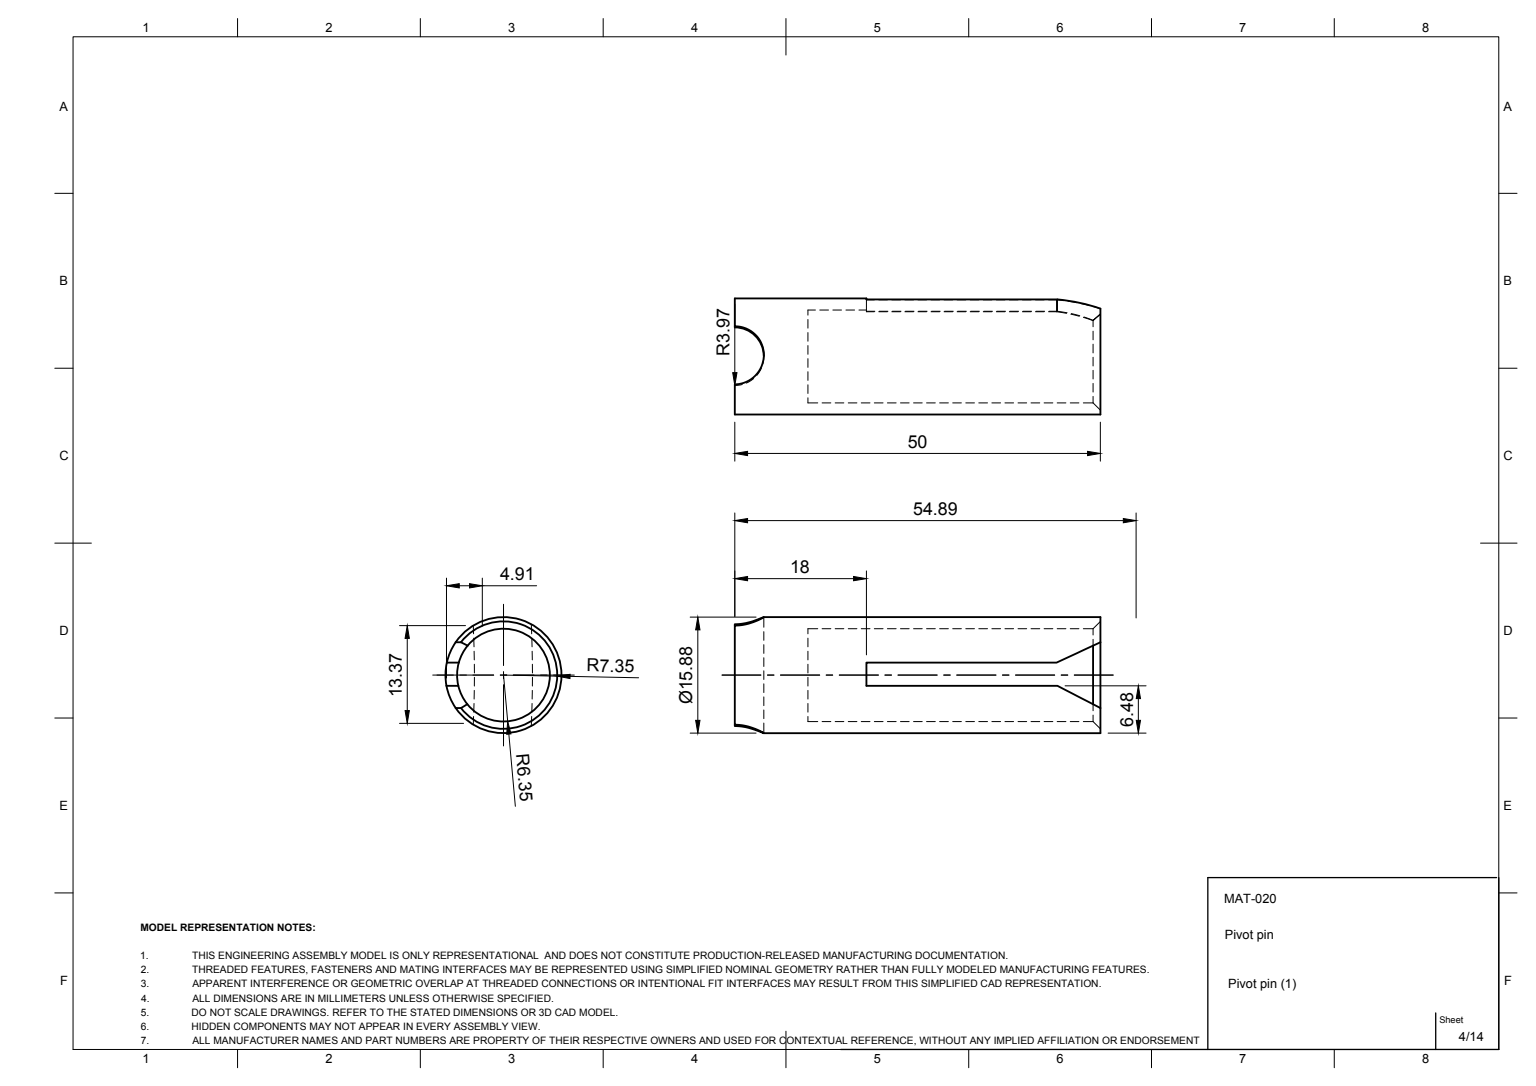
ISO-10303-21;
HEADER;
/* Generated by software containing ST-Developer
 * from STEP Tools, Inc. (www.steptools.com) 
 */

FILE_DESCRIPTION(
/* description */ ('STEP AP214'),
/* implementation_level */ '2;1');

FILE_NAME(
/* name */ 'Pivot Pin.step',
/* time_stamp */ '2026-11-14T06:20:50-08:00',
/* author */ (''),
/* organization */ (''),
/* preprocessor_version */ 'ST-DEVELOPER v20.2',
/* originating_system */ 'Autodesk Translation Framework v15.17.0.0',
/* authorisation */ '');

FILE_SCHEMA (('AUTOMOTIVE_DESIGN { 1 0 10303 214 3 1 1 }'));
ENDSEC;

DATA;
#10=MECHANICAL_DESIGN_GEOMETRIC_PRESENTATION_REPRESENTATION('',(#967),#20658);
#115=CONICAL_SURFACE('',#4073,6.35000000000001,0.785398163397456);
#148=ELLIPSE('',#4079,13.8289418104825,6.34999999998296);
#149=ELLIPSE('',#4080,15.0727020037017,6.35000000001005);
#150=ELLIPSE('',#4086,17.286177263089,7.93749999997138);
#151=ELLIPSE('',#4088,18.840877504683,7.93750000004892);
#292=(
BOUNDED_CURVE()
B_SPLINE_CURVE(2,(#20498,#20499,#20500),.UNSPECIFIED.,.F.,.F.)
B_SPLINE_CURVE_WITH_KNOTS((3,3),(0.0183343553427957,0.042559607390491),
 .UNSPECIFIED.)
CURVE()
GEOMETRIC_REPRESENTATION_ITEM()
RATIONAL_B_SPLINE_CURVE((1.12800823010849,1.2118132350172,1.29359962909812))
REPRESENTATION_ITEM('')
);
#293=(
BOUNDED_CURVE()
B_SPLINE_CURVE(2,(#20503,#20504,#20505),.UNSPECIFIED.,.F.,.F.)
B_SPLINE_CURVE_WITH_KNOTS((3,3),(-0.061743756665462,-0.0265578055647394),
 .UNSPECIFIED.)
CURVE()
GEOMETRIC_REPRESENTATION_ITEM()
RATIONAL_B_SPLINE_CURVE((1.28203378876711,1.20432016972132,1.12358878740287))
REPRESENTATION_ITEM('')
);
#391=B_SPLINE_CURVE_WITH_KNOTS('',3,(#20526,#20527,#20528,#20529,#20530,
#20531,#20532,#20533,#20534,#20535,#20536,#20537,#20538,#20539,#20540,#20541,
#20542,#20543,#20544,#20545,#20546,#20547),.UNSPECIFIED.,.F.,.F.,(4,2,2,
2,2,2,2,2,2,2,4),(1.27322512801248,1.33474273520392,1.47506259652504,1.63354487754016,
1.7891729428134,1.93308978701607,2.07370553081328,2.22765816465705,2.39186406247873,
2.46887047840366,2.54509076244393),.UNSPECIFIED.);
#392=B_SPLINE_CURVE_WITH_KNOTS('',3,(#20567,#20568,#20569,#20570,#20571,
#20572,#20573,#20574,#20575,#20576,#20577,#20578,#20579,#20580,#20581,#20582,
#20583,#20584,#20585,#20586),.UNSPECIFIED.,.F.,.F.,(4,2,2,2,2,2,2,2,2,4),
(0.,0.133781719517655,0.281821942641468,0.447759981880601,0.597114390464313,
0.737248938214622,0.881128826876862,1.04037144466368,1.19403526065854,1.27322512801215),
 .UNSPECIFIED.);
#439=PLANE('',#4091);
#440=PLANE('',#4093);
#441=PLANE('',#4095);
#442=PLANE('',#4096);
#443=PLANE('',#4097);
#444=PLANE('',#4098);
#445=PLANE('',#4099);
#446=PLANE('',#4100);
#447=PLANE('',#4102);
#629=LINE('',#20510,#822);
#630=LINE('',#20514,#823);
#631=LINE('',#20519,#824);
#632=LINE('',#20551,#825);
#633=LINE('',#20557,#826);
#634=LINE('',#20561,#827);
#635=LINE('',#20592,#828);
#636=LINE('',#20593,#829);
#637=LINE('',#20595,#830);
#638=LINE('',#20596,#831);
#639=LINE('',#20598,#832);
#640=LINE('',#20600,#833);
#822=VECTOR('',#4874,6.35000000000001);
#823=VECTOR('',#4877,1000.);
#824=VECTOR('',#4882,1000.);
#825=VECTOR('',#4891,7.93750000000001);
#826=VECTOR('',#4896,1000.);
#827=VECTOR('',#4899,1000.);
#828=VECTOR('',#4916,1000.);
#829=VECTOR('',#4917,1000.);
#830=VECTOR('',#4920,1000.);
#831=VECTOR('',#4921,1000.);
#832=VECTOR('',#4924,1000.);
#833=VECTOR('',#4927,1000.);
#930=CYLINDRICAL_SURFACE('',#4076,6.35000000000001);
#931=CYLINDRICAL_SURFACE('',#4082,7.93750000000001);
#943=SHAPE_REPRESENTATION_RELATIONSHIP('SRR','None',#20727,#955);
#955=ADVANCED_BREP_SHAPE_REPRESENTATION('',(#979),#20657);
#967=STYLED_ITEM('',(#20786),#979);
#979=MANIFOLD_SOLID_BREP('Body1',#3662);
#1176=FACE_OUTER_BOUND('',#1408,.T.);
#1177=FACE_OUTER_BOUND('',#1409,.T.);
#1178=FACE_OUTER_BOUND('',#1410,.T.);
#1179=FACE_OUTER_BOUND('',#1411,.T.);
#1180=FACE_OUTER_BOUND('',#1412,.T.);
#1181=FACE_OUTER_BOUND('',#1413,.T.);
#1182=FACE_OUTER_BOUND('',#1414,.T.);
#1183=FACE_OUTER_BOUND('',#1415,.T.);
#1184=FACE_OUTER_BOUND('',#1416,.T.);
#1185=FACE_OUTER_BOUND('',#1417,.T.);
#1186=FACE_OUTER_BOUND('',#1418,.T.);
#1187=FACE_OUTER_BOUND('',#1419,.T.);
#1188=FACE_OUTER_BOUND('',#1420,.T.);
#1408=EDGE_LOOP('',(#3374,#3375,#3376,#3377));
#1409=EDGE_LOOP('',(#3378,#3379,#3380,#3381,#3382,#3383,#3384,#3385,#3386,
#3387));
#1410=EDGE_LOOP('',(#3388,#3389,#3390,#3391,#3392,#3393,#3394,#3395,#3396,
#3397,#3398,#3399,#3400,#3401));
#1411=EDGE_LOOP('',(#3402,#3403,#3404));
#1412=EDGE_LOOP('',(#3405,#3406));
#1413=EDGE_LOOP('',(#3407,#3408,#3409,#3410,#3411));
#1414=EDGE_LOOP('',(#3412,#3413,#3414,#3415));
#1415=EDGE_LOOP('',(#3416,#3417,#3418,#3419,#3420));
#1416=EDGE_LOOP('',(#3421,#3422,#3423,#3424));
#1417=EDGE_LOOP('',(#3425,#3426,#3427,#3428,#3429));
#1418=EDGE_LOOP('',(#3430,#3431,#3432,#3433,#3434));
#1419=EDGE_LOOP('',(#3435,#3436,#3437,#3438));
#1420=EDGE_LOOP('',(#3439));
#1533=CIRCLE('',#4074,6.35000000000001);
#1534=CIRCLE('',#4075,7.35000000000003);
#1535=CIRCLE('',#4077,6.35000000000001);
#1536=CIRCLE('',#4078,6.35000000000001);
#1537=CIRCLE('',#4081,6.35000000000001);
#1538=CIRCLE('',#4083,7.93750000000001);
#1539=CIRCLE('',#4084,7.93750000000001);
#1540=CIRCLE('',#4085,7.93750000000001);
#1541=CIRCLE('',#4087,7.93750000000001);
#1542=CIRCLE('',#4089,7.93750000000001);
#1543=CIRCLE('',#4090,7.93750000000001);
#1544=CIRCLE('',#4092,153.96875);
#1545=CIRCLE('',#4094,146.03125);
#1861=VERTEX_POINT('',#20494);
#1862=VERTEX_POINT('',#20495);
#1863=VERTEX_POINT('',#20497);
#1864=VERTEX_POINT('',#20501);
#1865=VERTEX_POINT('',#20507);
#1866=VERTEX_POINT('',#20509);
#1867=VERTEX_POINT('',#20511);
#1868=VERTEX_POINT('',#20513);
#1869=VERTEX_POINT('',#20516);
#1870=VERTEX_POINT('',#20518);
#1871=VERTEX_POINT('',#20522);
#1872=VERTEX_POINT('',#20523);
#1873=VERTEX_POINT('',#20525);
#1874=VERTEX_POINT('',#20548);
#1875=VERTEX_POINT('',#20550);
#1876=VERTEX_POINT('',#20552);
#1877=VERTEX_POINT('',#20554);
#1878=VERTEX_POINT('',#20556);
#1879=VERTEX_POINT('',#20558);
#1880=VERTEX_POINT('',#20560);
#1881=VERTEX_POINT('',#20562);
#1882=VERTEX_POINT('',#20565);
#2369=EDGE_CURVE('',#1861,#1862,#1533,.T.);
#2370=EDGE_CURVE('',#1863,#1861,#292,.T.);
#2371=EDGE_CURVE('',#1864,#1863,#1534,.T.);
#2372=EDGE_CURVE('',#1862,#1864,#293,.T.);
#2373=EDGE_CURVE('',#1865,#1865,#1535,.T.);
#2374=EDGE_CURVE('',#1865,#1866,#629,.T.);
#2375=EDGE_CURVE('',#1867,#1866,#1536,.T.);
#2376=EDGE_CURVE('',#1868,#1867,#630,.T.);
#2377=EDGE_CURVE('',#1861,#1868,#148,.T.);
#2378=EDGE_CURVE('',#1869,#1862,#149,.T.);
#2379=EDGE_CURVE('',#1870,#1869,#631,.T.);
#2380=EDGE_CURVE('',#1866,#1870,#1537,.T.);
#2381=EDGE_CURVE('',#1871,#1872,#1538,.T.);
#2382=EDGE_CURVE('',#1872,#1873,#391,.T.);
#2383=EDGE_CURVE('',#1873,#1874,#1539,.T.);
#2384=EDGE_CURVE('',#1874,#1875,#632,.T.);
#2385=EDGE_CURVE('',#1876,#1875,#1540,.T.);
#2386=EDGE_CURVE('',#1876,#1877,#150,.T.);
#2387=EDGE_CURVE('',#1877,#1878,#633,.T.);
#2388=EDGE_CURVE('',#1878,#1879,#1541,.T.);
#2389=EDGE_CURVE('',#1879,#1880,#634,.T.);
#2390=EDGE_CURVE('',#1880,#1881,#151,.T.);
#2391=EDGE_CURVE('',#1875,#1881,#1542,.T.);
#2392=EDGE_CURVE('',#1874,#1882,#1543,.T.);
#2393=EDGE_CURVE('',#1882,#1871,#392,.T.);
#2394=EDGE_CURVE('',#1873,#1882,#1544,.T.);
#2395=EDGE_CURVE('',#1871,#1872,#1545,.T.);
#2396=EDGE_CURVE('',#1864,#1881,#635,.T.);
#2397=EDGE_CURVE('',#1876,#1863,#636,.T.);
#2398=EDGE_CURVE('',#1879,#1870,#637,.T.);
#2399=EDGE_CURVE('',#1880,#1869,#638,.T.);
#2400=EDGE_CURVE('',#1878,#1867,#639,.T.);
#2401=EDGE_CURVE('',#1877,#1868,#640,.T.);
#3374=ORIENTED_EDGE('',*,*,#2369,.F.);
#3375=ORIENTED_EDGE('',*,*,#2370,.F.);
#3376=ORIENTED_EDGE('',*,*,#2371,.F.);
#3377=ORIENTED_EDGE('',*,*,#2372,.F.);
#3378=ORIENTED_EDGE('',*,*,#2373,.F.);
#3379=ORIENTED_EDGE('',*,*,#2374,.T.);
#3380=ORIENTED_EDGE('',*,*,#2375,.F.);
#3381=ORIENTED_EDGE('',*,*,#2376,.F.);
#3382=ORIENTED_EDGE('',*,*,#2377,.F.);
#3383=ORIENTED_EDGE('',*,*,#2369,.T.);
#3384=ORIENTED_EDGE('',*,*,#2378,.F.);
#3385=ORIENTED_EDGE('',*,*,#2379,.F.);
#3386=ORIENTED_EDGE('',*,*,#2380,.F.);
#3387=ORIENTED_EDGE('',*,*,#2374,.F.);
#3388=ORIENTED_EDGE('',*,*,#2381,.T.);
#3389=ORIENTED_EDGE('',*,*,#2382,.T.);
#3390=ORIENTED_EDGE('',*,*,#2383,.T.);
#3391=ORIENTED_EDGE('',*,*,#2384,.T.);
#3392=ORIENTED_EDGE('',*,*,#2385,.F.);
#3393=ORIENTED_EDGE('',*,*,#2386,.T.);
#3394=ORIENTED_EDGE('',*,*,#2387,.T.);
#3395=ORIENTED_EDGE('',*,*,#2388,.T.);
#3396=ORIENTED_EDGE('',*,*,#2389,.T.);
#3397=ORIENTED_EDGE('',*,*,#2390,.T.);
#3398=ORIENTED_EDGE('',*,*,#2391,.F.);
#3399=ORIENTED_EDGE('',*,*,#2384,.F.);
#3400=ORIENTED_EDGE('',*,*,#2392,.T.);
#3401=ORIENTED_EDGE('',*,*,#2393,.T.);
#3402=ORIENTED_EDGE('',*,*,#2394,.T.);
#3403=ORIENTED_EDGE('',*,*,#2392,.F.);
#3404=ORIENTED_EDGE('',*,*,#2383,.F.);
#3405=ORIENTED_EDGE('',*,*,#2395,.T.);
#3406=ORIENTED_EDGE('',*,*,#2381,.F.);
#3407=ORIENTED_EDGE('',*,*,#2396,.F.);
#3408=ORIENTED_EDGE('',*,*,#2371,.T.);
#3409=ORIENTED_EDGE('',*,*,#2397,.F.);
#3410=ORIENTED_EDGE('',*,*,#2385,.T.);
#3411=ORIENTED_EDGE('',*,*,#2391,.T.);
#3412=ORIENTED_EDGE('',*,*,#2398,.T.);
#3413=ORIENTED_EDGE('',*,*,#2379,.T.);
#3414=ORIENTED_EDGE('',*,*,#2399,.F.);
#3415=ORIENTED_EDGE('',*,*,#2389,.F.);
#3416=ORIENTED_EDGE('',*,*,#2400,.T.);
#3417=ORIENTED_EDGE('',*,*,#2375,.T.);
#3418=ORIENTED_EDGE('',*,*,#2380,.T.);
#3419=ORIENTED_EDGE('',*,*,#2398,.F.);
#3420=ORIENTED_EDGE('',*,*,#2388,.F.);
#3421=ORIENTED_EDGE('',*,*,#2401,.T.);
#3422=ORIENTED_EDGE('',*,*,#2376,.T.);
#3423=ORIENTED_EDGE('',*,*,#2400,.F.);
#3424=ORIENTED_EDGE('',*,*,#2387,.F.);
#3425=ORIENTED_EDGE('',*,*,#2397,.T.);
#3426=ORIENTED_EDGE('',*,*,#2370,.T.);
#3427=ORIENTED_EDGE('',*,*,#2377,.T.);
#3428=ORIENTED_EDGE('',*,*,#2401,.F.);
#3429=ORIENTED_EDGE('',*,*,#2386,.F.);
#3430=ORIENTED_EDGE('',*,*,#2378,.T.);
#3431=ORIENTED_EDGE('',*,*,#2372,.T.);
#3432=ORIENTED_EDGE('',*,*,#2396,.T.);
#3433=ORIENTED_EDGE('',*,*,#2390,.F.);
#3434=ORIENTED_EDGE('',*,*,#2399,.T.);
#3435=ORIENTED_EDGE('',*,*,#2395,.F.);
#3436=ORIENTED_EDGE('',*,*,#2393,.F.);
#3437=ORIENTED_EDGE('',*,*,#2394,.F.);
#3438=ORIENTED_EDGE('',*,*,#2382,.F.);
#3439=ORIENTED_EDGE('',*,*,#2373,.T.);
#3441=TOROIDAL_SURFACE('',#4101,150.,3.96875);
#3638=ADVANCED_FACE('',(#1176),#115,.F.);
#3639=ADVANCED_FACE('',(#1177),#930,.F.);
#3640=ADVANCED_FACE('',(#1178),#931,.T.);
#3641=ADVANCED_FACE('',(#1179),#439,.F.);
#3642=ADVANCED_FACE('',(#1180),#440,.F.);
#3643=ADVANCED_FACE('',(#1181),#441,.T.);
#3644=ADVANCED_FACE('',(#1182),#442,.F.);
#3645=ADVANCED_FACE('',(#1183),#443,.F.);
#3646=ADVANCED_FACE('',(#1184),#444,.F.);
#3647=ADVANCED_FACE('',(#1185),#445,.F.);
#3648=ADVANCED_FACE('',(#1186),#446,.F.);
#3649=ADVANCED_FACE('',(#1187),#3441,.F.);
#3650=ADVANCED_FACE('',(#1188),#447,.T.);
#3662=CLOSED_SHELL('',(#3638,#3639,#3640,#3641,#3642,#3643,#3644,#3645,
#3646,#3647,#3648,#3649,#3650));
#4072=AXIS2_PLACEMENT_3D('',#20492,#4862,#4863);
#4073=AXIS2_PLACEMENT_3D('',#20493,#4864,#4865);
#4074=AXIS2_PLACEMENT_3D('',#20496,#4866,#4867);
#4075=AXIS2_PLACEMENT_3D('',#20502,#4868,#4869);
#4076=AXIS2_PLACEMENT_3D('',#20506,#4870,#4871);
#4077=AXIS2_PLACEMENT_3D('',#20508,#4872,#4873);
#4078=AXIS2_PLACEMENT_3D('',#20512,#4875,#4876);
#4079=AXIS2_PLACEMENT_3D('',#20515,#4878,#4879);
#4080=AXIS2_PLACEMENT_3D('',#20517,#4880,#4881);
#4081=AXIS2_PLACEMENT_3D('',#20520,#4883,#4884);
#4082=AXIS2_PLACEMENT_3D('',#20521,#4885,#4886);
#4083=AXIS2_PLACEMENT_3D('',#20524,#4887,#4888);
#4084=AXIS2_PLACEMENT_3D('',#20549,#4889,#4890);
#4085=AXIS2_PLACEMENT_3D('',#20553,#4892,#4893);
#4086=AXIS2_PLACEMENT_3D('',#20555,#4894,#4895);
#4087=AXIS2_PLACEMENT_3D('',#20559,#4897,#4898);
#4088=AXIS2_PLACEMENT_3D('',#20563,#4900,#4901);
#4089=AXIS2_PLACEMENT_3D('',#20564,#4902,#4903);
#4090=AXIS2_PLACEMENT_3D('',#20566,#4904,#4905);
#4091=AXIS2_PLACEMENT_3D('',#20587,#4906,#4907);
#4092=AXIS2_PLACEMENT_3D('',#20588,#4908,#4909);
#4093=AXIS2_PLACEMENT_3D('',#20589,#4910,#4911);
#4094=AXIS2_PLACEMENT_3D('',#20590,#4912,#4913);
#4095=AXIS2_PLACEMENT_3D('',#20591,#4914,#4915);
#4096=AXIS2_PLACEMENT_3D('',#20594,#4918,#4919);
#4097=AXIS2_PLACEMENT_3D('',#20597,#4922,#4923);
#4098=AXIS2_PLACEMENT_3D('',#20599,#4925,#4926);
#4099=AXIS2_PLACEMENT_3D('',#20601,#4928,#4929);
#4100=AXIS2_PLACEMENT_3D('',#20602,#4930,#4931);
#4101=AXIS2_PLACEMENT_3D('',#20603,#4932,#4933);
#4102=AXIS2_PLACEMENT_3D('',#20604,#4934,#4935);
#4862=DIRECTION('axis',(0.,0.,1.));
#4863=DIRECTION('refdir',(1.,0.,0.));
#4864=DIRECTION('center_axis',(0.,1.,0.));
#4865=DIRECTION('ref_axis',(0.,0.,1.));
#4866=DIRECTION('center_axis',(0.,1.,0.));
#4867=DIRECTION('ref_axis',(0.,0.,1.));
#4868=DIRECTION('center_axis',(0.,-1.,0.));
#4869=DIRECTION('ref_axis',(0.,0.,1.));
#4870=DIRECTION('center_axis',(0.,1.,0.));
#4871=DIRECTION('ref_axis',(0.,0.,1.));
#4872=DIRECTION('center_axis',(0.,1.,0.));
#4873=DIRECTION('ref_axis',(0.,0.,1.));
#4874=DIRECTION('',(0.,1.,0.));
#4875=DIRECTION('center_axis',(0.,-1.,0.));
#4876=DIRECTION('ref_axis',(0.,0.,-1.));
#4877=DIRECTION('',(0.,-1.,0.));
#4878=DIRECTION('center_axis',(-0.888342258257525,-0.459181916231379,-4.393783563666E-14));
#4879=DIRECTION('ref_axis',(0.459181916231379,-0.888342258257525,-4.20136709809981E-13));
#4880=DIRECTION('center_axis',(0.906925322797953,-0.42129141798502,3.93873602430886E-13));
#4881=DIRECTION('ref_axis',(0.42129141798502,0.906925322797953,-2.61951590649629E-13));
#4882=DIRECTION('',(0.,1.,0.));
#4883=DIRECTION('center_axis',(0.,-1.,0.));
#4884=DIRECTION('ref_axis',(0.,0.,-1.));
#4885=DIRECTION('center_axis',(0.,-1.,0.));
#4886=DIRECTION('ref_axis',(0.,0.,-1.));
#4887=DIRECTION('center_axis',(0.,1.,0.));
#4888=DIRECTION('ref_axis',(0.,0.,1.));
#4889=DIRECTION('center_axis',(0.,1.,0.));
#4890=DIRECTION('ref_axis',(0.,0.,1.));
#4891=DIRECTION('',(0.,1.,0.));
#4892=DIRECTION('center_axis',(0.,1.,0.));
#4893=DIRECTION('ref_axis',(0.,0.,1.));
#4894=DIRECTION('center_axis',(-0.888342258257544,-0.459181916231341,-3.75501605328633E-13));
#4895=DIRECTION('ref_axis',(0.459181916231341,-0.888342258257545,-8.50644926987111E-13));
#4896=DIRECTION('',(0.,-1.,0.));
#4897=DIRECTION('center_axis',(0.,-1.,0.));
#4898=DIRECTION('ref_axis',(0.,0.,-1.));
#4899=DIRECTION('',(0.,1.,0.));
#4900=DIRECTION('center_axis',(0.906925322797957,-0.421291417985012,2.87289631591583E-13));
#4901=DIRECTION('ref_axis',(0.421291417985012,0.906925322797957,-1.29853851007989E-12));
#4902=DIRECTION('center_axis',(0.,1.,0.));
#4903=DIRECTION('ref_axis',(0.,0.,1.));
#4904=DIRECTION('center_axis',(0.,1.,0.));
#4905=DIRECTION('ref_axis',(0.,0.,1.));
#4906=DIRECTION('center_axis',(0.,1.,0.));
#4907=DIRECTION('ref_axis',(0.,0.,1.));
#4908=DIRECTION('center_axis',(0.,1.,0.));
#4909=DIRECTION('ref_axis',(0.,0.,1.));
#4910=DIRECTION('center_axis',(0.,1.,0.));
#4911=DIRECTION('ref_axis',(0.,0.,1.));
#4912=DIRECTION('center_axis',(0.,-1.,0.));
#4913=DIRECTION('ref_axis',(0.,0.,-1.));
#4914=DIRECTION('center_axis',(0.,1.,0.));
#4915=DIRECTION('ref_axis',(0.,0.,1.));
#4916=DIRECTION('',(0.,0.,-1.));
#4917=DIRECTION('',(0.,0.,1.));
#4918=DIRECTION('center_axis',(1.,0.,0.));
#4919=DIRECTION('ref_axis',(0.,0.,-1.));
#4920=DIRECTION('',(0.,0.,1.));
#4921=DIRECTION('',(0.,0.,1.));
#4922=DIRECTION('center_axis',(0.,-1.,0.));
#4923=DIRECTION('ref_axis',(0.,0.,-1.));
#4924=DIRECTION('',(0.,0.,1.));
#4925=DIRECTION('center_axis',(-1.,-1.16210731118036E-16,-1.36736175538941E-63));
#4926=DIRECTION('ref_axis',(1.16210731118036E-16,-1.,-6.16297582203915E-33));
#4927=DIRECTION('',(0.,0.,1.));
#4928=DIRECTION('center_axis',(-0.888342258257513,-0.459181916231401,1.66533453693773E-16));
#4929=DIRECTION('ref_axis',(0.459181916231401,-0.888342258257513,-9.95253396589023E-33));
#4930=DIRECTION('center_axis',(0.906925322797977,-0.421291417984968,5.55111512312578E-17));
#4931=DIRECTION('ref_axis',(0.421291417984968,0.906925322797977,2.77555756156289E-17));
#4932=DIRECTION('center_axis',(0.,1.,0.));
#4933=DIRECTION('ref_axis',(1.,0.,1.03372647248395E-14));
#4934=DIRECTION('center_axis',(0.,1.,0.));
#4935=DIRECTION('ref_axis',(0.,0.,1.));
#20492=CARTESIAN_POINT('',(0.,0.,0.));
#20493=CARTESIAN_POINT('Origin',(0.,49.,0.));
#20494=CARTESIAN_POINT('',(-3.98310247321554,49.,-4.94544180916756));
#20495=CARTESIAN_POINT('',(4.03547286927067,49.,-4.90280110971059));
#20496=CARTESIAN_POINT('Origin',(0.,49.,0.));
#20497=CARTESIAN_POINT('',(-4.5,50.,-5.81141118834299));
#20498=CARTESIAN_POINT('Ctrl Pts',(-4.49999999999977,49.9999999999993,-5.81141118834253));
#20499=CARTESIAN_POINT('Ctrl Pts',(-4.22074508491678,49.4597480146199,-5.34436370422895));
#20500=CARTESIAN_POINT('Ctrl Pts',(-3.98310247321565,48.9999999999999,-4.94544180916757));
#20501=CARTESIAN_POINT('',(4.50000000000003,50.,-5.8114111883431));
#20502=CARTESIAN_POINT('Origin',(0.,50.,0.));
#20503=CARTESIAN_POINT('Ctrl Pts',(4.03547286927078,49.,-4.90280110971056));
#20504=CARTESIAN_POINT('Ctrl Pts',(4.24803951147274,49.4575979057849,-5.32050921950116));
#20505=CARTESIAN_POINT('Ctrl Pts',(4.50000000000141,50.0000000000031,-5.81141118834603));
#20506=CARTESIAN_POINT('Origin',(0.,10.,0.));
#20507=CARTESIAN_POINT('',(-7.7765071745857E-16,10.,-6.35000000000001));
#20508=CARTESIAN_POINT('Origin',(0.,10.,0.));
#20509=CARTESIAN_POINT('',(-7.7765071745857E-16,18.,-6.35000000000001));
#20510=CARTESIAN_POINT('',(-7.7765071745857E-16,10.,-6.35000000000001));
#20511=CARTESIAN_POINT('',(-1.46216278437505,18.,-6.17936728087826));
#20512=CARTESIAN_POINT('Origin',(0.,18.,0.));
#20513=CARTESIAN_POINT('',(-1.46216278437505,44.122941089459,-6.17936728087826));
#20514=CARTESIAN_POINT('',(-1.46216278437505,10.,-6.17936728087826));
#20515=CARTESIAN_POINT('Origin',(-5.47117906535277E-12,41.2942125531358,
-1.69803060501295E-11));
#20516=CARTESIAN_POINT('',(1.71283721562501,44.,-6.11462907074245));
#20517=CARTESIAN_POINT('Origin',(-4.41341407864115E-12,40.3127294353338,
1.04150021940086E-11));
#20518=CARTESIAN_POINT('',(1.71283721562501,18.,-6.11462907074245));
#20519=CARTESIAN_POINT('',(1.71283721562501,10.,-6.11462907074245));
#20520=CARTESIAN_POINT('Origin',(0.,18.,0.));
#20521=CARTESIAN_POINT('Origin',(0.,50.,0.));
#20522=CARTESIAN_POINT('',(6.78069956542715,0.,-4.12625976562492));
#20523=CARTESIAN_POINT('',(-6.78069956542721,0.,-4.12625976562492));
#20524=CARTESIAN_POINT('Origin',(0.,0.,0.));
#20525=CARTESIAN_POINT('',(-6.96263988196173,-2.54796184151473E-11,3.81124023437512));
#20526=CARTESIAN_POINT('Ctrl Pts',(-6.78069956542709,-1.59594559789866E-15,
-4.12625976562516));
#20527=CARTESIAN_POINT('Ctrl Pts',(-6.78069956542709,0.20291602635612,-4.12625976562516));
#20528=CARTESIAN_POINT('Ctrl Pts',(-6.789971315478,0.40609151683513,-4.11113887165097));
#20529=CARTESIAN_POINT('Ctrl Pts',(-6.85001139901333,1.06933946691968,-4.01096526257536));
#20530=CARTESIAN_POINT('Ctrl Pts',(-6.93780786854016,1.50828047099799,-3.8638114398035));
#20531=CARTESIAN_POINT('Ctrl Pts',(-7.17422155741041,2.36061047309084,-3.40717387141783));
#20532=CARTESIAN_POINT('Ctrl Pts',(-7.32703301852759,2.75937873020496,-3.08105830459423));
#20533=CARTESIAN_POINT('Ctrl Pts',(-7.60736246330475,3.40131175443517,-2.3022040118231));
#20534=CARTESIAN_POINT('Ctrl Pts',(-7.73374530365473,3.64481097932461,-1.85477666749764));
#20535=CARTESIAN_POINT('Ctrl Pts',(-7.89829313943706,3.93499941473798,-0.912243104787409));
#20536=CARTESIAN_POINT('Ctrl Pts',(-7.93998719122528,3.99124892394717,-0.436363089125317));
#20537=CARTESIAN_POINT('Ctrl Pts',(-7.93483838332232,3.9308187778951,0.511588998034206));
#20538=CARTESIAN_POINT('Ctrl Pts',(-7.89016948894505,3.81908070047316,0.967194108666593));
#20539=CARTESIAN_POINT('Ctrl Pts',(-7.73156920749371,3.43283541545737,1.85744415264528));
#20540=CARTESIAN_POINT('Ctrl Pts',(-7.6131090943576,3.1475122718246,2.27716767192686));
#20541=CARTESIAN_POINT('Ctrl Pts',(-7.35583080822277,2.42434696900374,3.00933293642248));
#20542=CARTESIAN_POINT('Ctrl Pts',(-7.21682951488633,1.97770824086303,3.31262246589732));
#20543=CARTESIAN_POINT('Ctrl Pts',(-7.06811858761907,1.24745024754987,3.61345869274962));
#20544=CARTESIAN_POINT('Ctrl Pts',(-7.02926529552173,1.00441501289051,3.68734467939022));
#20545=CARTESIAN_POINT('Ctrl Pts',(-6.97647739981983,0.506199451376457,
3.7862620052672));
#20546=CARTESIAN_POINT('Ctrl Pts',(-6.96263988196164,0.254067613467043,
3.81124023437485));
#20547=CARTESIAN_POINT('Ctrl Pts',(-6.96263988196164,0.,3.81124023437485));
#20548=CARTESIAN_POINT('',(-9.72063396823213E-16,0.,7.93750000000001));
#20549=CARTESIAN_POINT('Origin',(0.,0.,0.));
#20550=CARTESIAN_POINT('',(-9.72063396823213E-16,50.,7.93750000000001));
#20551=CARTESIAN_POINT('',(-9.72063396823213E-16,50.,7.93750000000001));
#20552=CARTESIAN_POINT('',(-4.50000000000012,50.,-6.53864712689098));
#20553=CARTESIAN_POINT('Origin',(0.,50.,0.));
#20554=CARTESIAN_POINT('',(-1.46216278437508,44.122941089459,-7.80166560690648));
#20555=CARTESIAN_POINT('Origin',(-1.63441482570192E-11,41.2942125531507,
-2.83206791351631E-11));
#20556=CARTESIAN_POINT('',(-1.46216278437508,18.,-7.80166560690648));
#20557=CARTESIAN_POINT('',(-1.46216278437508,50.,-7.80166560690648));
#20558=CARTESIAN_POINT('',(1.71283721562494,18.,-7.75048997952832));
#20559=CARTESIAN_POINT('Origin',(0.,18.,0.));
#20560=CARTESIAN_POINT('',(1.71283721562494,44.,-7.75048997952832));
#20561=CARTESIAN_POINT('',(1.71283721562494,50.,-7.75048997952832));
#20562=CARTESIAN_POINT('',(4.49999999999992,50.,-6.53864712689095));
#20563=CARTESIAN_POINT('Origin',(-2.26108021195159E-11,40.3127294352942,
4.90707474654073E-11));
#20564=CARTESIAN_POINT('Origin',(0.,50.,0.));
#20565=CARTESIAN_POINT('',(6.96263988196147,0.,3.81124023437518));
#20566=CARTESIAN_POINT('Origin',(0.,0.,0.));
#20567=CARTESIAN_POINT('Ctrl Pts',(6.96263988196154,9.71445146547012E-16,
3.81124023437498));
#20568=CARTESIAN_POINT('Ctrl Pts',(6.96263988196154,0.445939065058851,3.81124023437498));
#20569=CARTESIAN_POINT('Ctrl Pts',(7.00600256018719,0.882552917010117,3.7345501133779));
#20570=CARTESIAN_POINT('Ctrl Pts',(7.16255453367982,1.7545618554345,3.42561203152615));
#20571=CARTESIAN_POINT('Ctrl Pts',(7.27981347983279,2.17438418007477,3.18093762861799));
#20572=CARTESIAN_POINT('Ctrl Pts',(7.53445421285187,2.94715506316683,2.52473565447381));
#20573=CARTESIAN_POINT('Ctrl Pts',(7.67173489201974,3.28625881372763,2.09625272246473));
#20574=CARTESIAN_POINT('Ctrl Pts',(7.8629249241042,3.75334095385897,1.17367468316625));
#20575=CARTESIAN_POINT('Ctrl Pts',(7.92235190096679,3.8959552204152,0.697053670144953));
#20576=CARTESIAN_POINT('Ctrl Pts',(7.94675012447075,3.99568166692586,-0.263277261294666));
#20577=CARTESIAN_POINT('Ctrl Pts',(7.91694647191713,3.96207512102207,-0.729006144604749));
#20578=CARTESIAN_POINT('Ctrl Pts',(7.78063473675749,3.73138702283732,-1.63778832271464));
#20579=CARTESIAN_POINT('Ctrl Pts',(7.67434248237991,3.53338352035958,-2.06587018517267));
#20580=CARTESIAN_POINT('Ctrl Pts',(7.41513175825483,2.9732220006111,-2.86618920547352));
#20581=CARTESIAN_POINT('Ctrl Pts',(7.26011037168438,2.59860363725,-3.22317703114952));
#20582=CARTESIAN_POINT('Ctrl Pts',(6.99433349067142,1.74884021981955,-3.76442418449406));
#20583=CARTESIAN_POINT('Ctrl Pts',(6.88384000315192,1.27946736789922,-3.95341867708105));
#20584=CARTESIAN_POINT('Ctrl Pts',(6.79611754991714,0.521986131736863,-4.10123268100205));
#20585=CARTESIAN_POINT('Ctrl Pts',(6.78069956542718,0.261208033678902,-4.12625976562502));
#20586=CARTESIAN_POINT('Ctrl Pts',(6.78069956542718,1.56125112837913E-16,
-4.12625976562502));
#20587=CARTESIAN_POINT('Origin',(0.,0.,0.));
#20588=CARTESIAN_POINT('Origin',(1.51267887105178E-12,0.,-150.));
#20589=CARTESIAN_POINT('Origin',(0.,0.,0.));
#20590=CARTESIAN_POINT('Origin',(1.51267887105178E-12,0.,-150.));
#20591=CARTESIAN_POINT('Origin',(0.,50.,0.));
#20592=CARTESIAN_POINT('',(4.49999999999989,50.,5.20417042793042E-14));
#20593=CARTESIAN_POINT('',(-4.50000000000012,50.,1.14491749414469E-13));
#20594=CARTESIAN_POINT('Origin',(1.71283721562496,18.,-40.0000000000001));
#20595=CARTESIAN_POINT('',(1.71283721562496,18.,-40.0000000000001));
#20596=CARTESIAN_POINT('',(1.71283721562496,44.,-40.0000000000001));
#20597=CARTESIAN_POINT('Origin',(-1.46216278437511,18.,-40.));
#20598=CARTESIAN_POINT('',(-1.46216278437511,18.,-40.));
#20599=CARTESIAN_POINT('Origin',(-1.46216278437511,44.122941089459,-40.));
#20600=CARTESIAN_POINT('',(-1.46216278437511,44.122941089459,-40.));
#20601=CARTESIAN_POINT('Origin',(-4.50000000000012,50.,-40.));
#20602=CARTESIAN_POINT('Origin',(1.71283721562496,44.,-40.0000000000001));
#20603=CARTESIAN_POINT('Origin',(1.51267887105178E-12,0.,-150.));
#20604=CARTESIAN_POINT('Origin',(0.,10.,0.));
#20643=UNCERTAINTY_MEASURE_WITH_UNIT(LENGTH_MEASURE(0.01),#20659,
'DISTANCE_ACCURACY_VALUE',
'Maximum model space distance between geometric entities at asserted c
onnectivities');
#20644=UNCERTAINTY_MEASURE_WITH_UNIT(LENGTH_MEASURE(0.01),#20659,
'DISTANCE_ACCURACY_VALUE',
'Maximum model space distance between geometric entities at asserted c
onnectivities');
#20657=(
GEOMETRIC_REPRESENTATION_CONTEXT(3)
GLOBAL_UNCERTAINTY_ASSIGNED_CONTEXT((#20643))
GLOBAL_UNIT_ASSIGNED_CONTEXT((#20659,#20661,#20662))
REPRESENTATION_CONTEXT('','3D')
);
#20658=(
GEOMETRIC_REPRESENTATION_CONTEXT(3)
GLOBAL_UNCERTAINTY_ASSIGNED_CONTEXT((#20644))
GLOBAL_UNIT_ASSIGNED_CONTEXT((#20659,#20661,#20662))
REPRESENTATION_CONTEXT('','3D')
);
#20659=(
LENGTH_UNIT()
NAMED_UNIT(*)
SI_UNIT(.MILLI.,.METRE.)
);
#20661=(
NAMED_UNIT(*)
PLANE_ANGLE_UNIT()
SI_UNIT($,.RADIAN.)
);
#20662=(
NAMED_UNIT(*)
SI_UNIT($,.STERADIAN.)
SOLID_ANGLE_UNIT()
);
#20675=SHAPE_DEFINITION_REPRESENTATION(#20688,#20727);
#20688=PRODUCT_DEFINITION_SHAPE('',$,#20741);
#20727=SHAPE_REPRESENTATION('',(#4072),#20657);
#20728=PRODUCT_DEFINITION_CONTEXT('part definition',#20769,'design');
#20741=PRODUCT_DEFINITION('Pivot pin','Pivot Pin',#20754,#20728);
#20754=PRODUCT_DEFINITION_FORMATION('',$,#20783);
#20769=APPLICATION_CONTEXT(
'Core Data for Automotive Mechanical Design Process');
#20770=PRODUCT_CONTEXT('part definition',#20769,'mechanical');
#20783=PRODUCT('Pivot pin','Pivot Pin','Pivot pin',(#20770));
#20786=PRESENTATION_STYLE_ASSIGNMENT((#20791));
#20791=SURFACE_STYLE_USAGE(.BOTH.,#20796);
#20796=SURFACE_SIDE_STYLE('',(#20801));
#20801=SURFACE_STYLE_FILL_AREA(#20806);
#20806=FILL_AREA_STYLE('Opaque(61,176,222)',(#20811));
#20811=FILL_AREA_STYLE_COLOUR('Opaque(61,176,222)',#20816);
#20816=COLOUR_RGB('Opaque(61,176,222)',0.23921568627451,0.690196078431373,
0.870588235294118);
ENDSEC;
END-ISO-10303-21;
